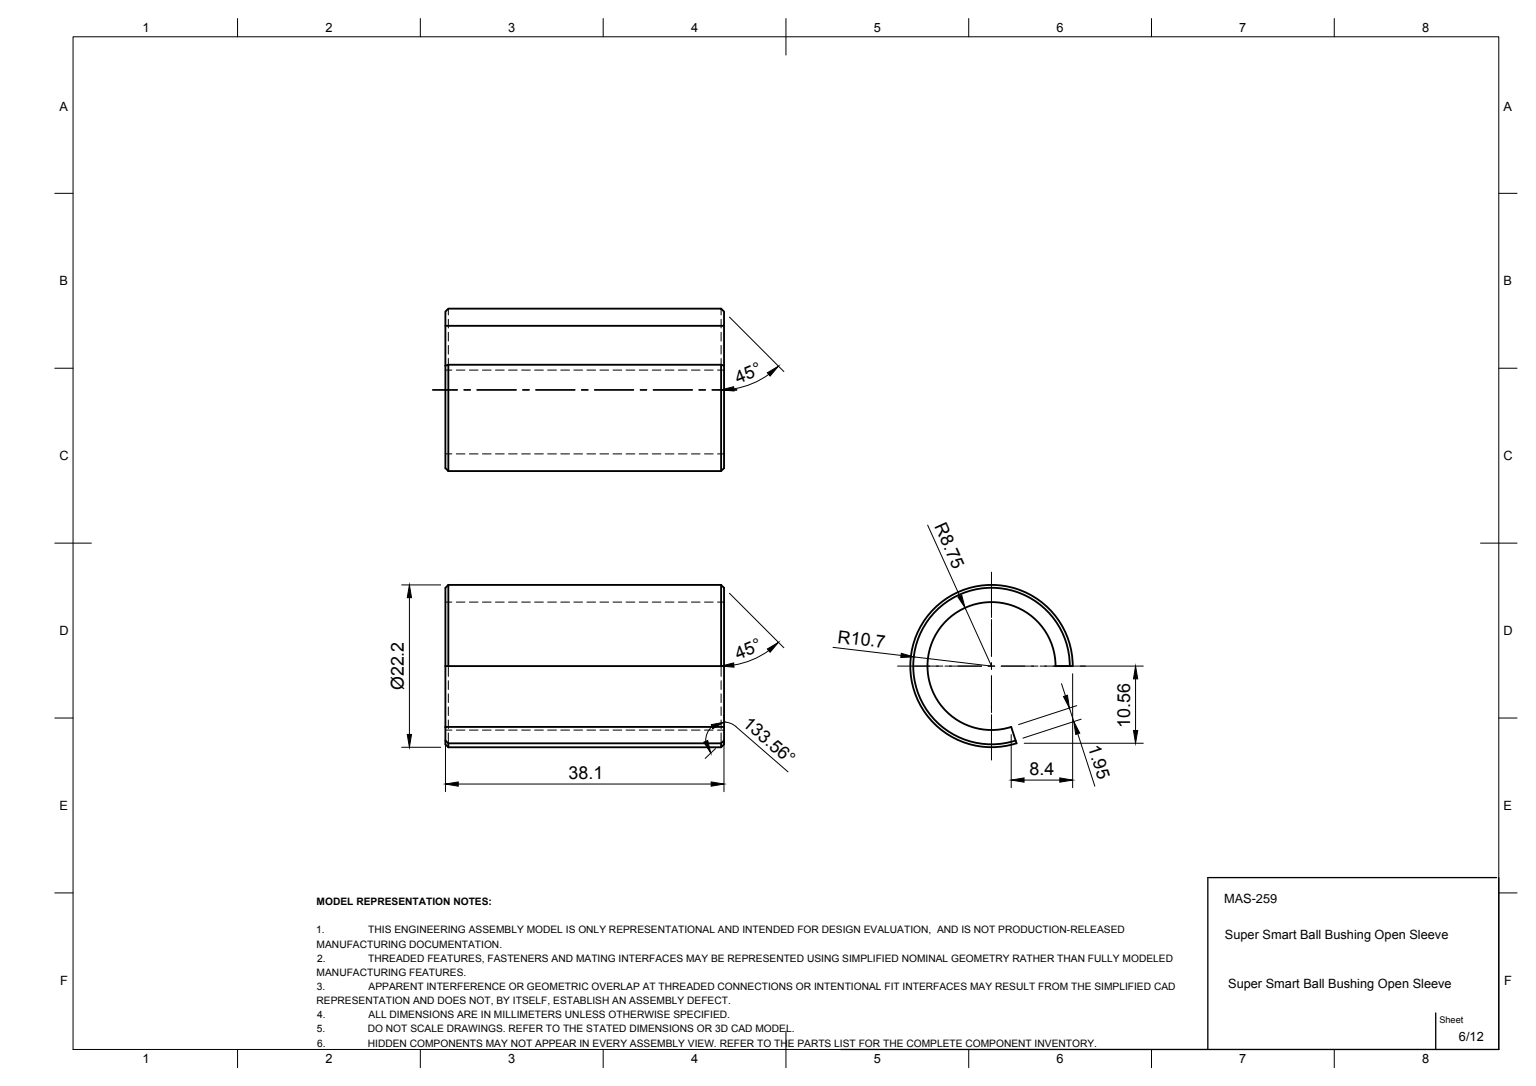
ISO-10303-21;
HEADER;
/* Generated by software containing ST-Developer
 * from STEP Tools, Inc. (www.steptools.com) 
 */

FILE_DESCRIPTION(
/* description */ (''),
/* implementation_level */ '2;1');

FILE_NAME(
/* name */ 'Super Smart Ball Bushing Open Sleeve.step',
/* time_stamp */ '2026-10-15T13:30:17-07:00',
/* author */ (''),
/* organization */ (''),
/* preprocessor_version */ 'ST-DEVELOPER v20.2',
/* originating_system */ 'Autodesk Translation Framework v15.15.0.0',
/* authorisation */ '');

FILE_SCHEMA (('AUTOMOTIVE_DESIGN { 1 0 10303 214 3 1 1 }'));
ENDSEC;

DATA;
#10=MECHANICAL_DESIGN_GEOMETRIC_PRESENTATION_REPRESENTATION('',(#1037),#71795);
#1017=SHAPE_REPRESENTATION_RELATIONSHIP('SRR','None',#72021,#1027);
#1027=ADVANCED_BREP_SHAPE_REPRESENTATION('',(#1047),#71789);
#1037=STYLED_ITEM('',(#72080),#1047);
#1047=MANIFOLD_SOLID_BREP('Body1',#13639);
#1092=CONICAL_SURFACE('',#14048,10.9,0.785398163397437);
#1093=CONICAL_SURFACE('',#14057,10.9,0.785398163397448);
#1624=PLANE('',#14046);
#1625=PLANE('',#14047);
#1626=PLANE('',#14051);
#1627=PLANE('',#14055);
#2178=FACE_OUTER_BOUND('',#2891,.T.);
#2179=FACE_OUTER_BOUND('',#2892,.T.);
#2180=FACE_OUTER_BOUND('',#2893,.T.);
#2181=FACE_OUTER_BOUND('',#2894,.T.);
#2182=FACE_OUTER_BOUND('',#2895,.T.);
#2183=FACE_OUTER_BOUND('',#2896,.T.);
#2184=FACE_OUTER_BOUND('',#2897,.T.);
#2185=FACE_OUTER_BOUND('',#2898,.T.);
#2891=EDGE_LOOP('',(#9677,#9678,#9679,#9680,#9681,#9682));
#2892=EDGE_LOOP('',(#9683,#9684,#9685,#9686,#9687,#9688));
#2893=EDGE_LOOP('',(#9689,#9690,#9691,#9692));
#2894=EDGE_LOOP('',(#9693,#9694,#9695,#9696));
#2895=EDGE_LOOP('',(#9697,#9698,#9699,#9700));
#2896=EDGE_LOOP('',(#9701,#9702,#9703,#9704));
#2897=EDGE_LOOP('',(#9705,#9706,#9707,#9708));
#2898=EDGE_LOOP('',(#9709,#9710,#9711,#9712));
#3531=CIRCLE('',#14049,10.7);
#3532=CIRCLE('',#14050,11.1);
#3533=CIRCLE('',#14052,8.75);
#3534=CIRCLE('',#14054,8.75);
#3535=CIRCLE('',#14056,10.7);
#3536=CIRCLE('',#14058,11.1);
#4023=LINE('',#19704,#4934);
#4024=LINE('',#19706,#4935);
#4025=LINE('',#19708,#4936);
#4026=LINE('',#19710,#4937);
#4027=LINE('',#19712,#4938);
#4028=LINE('',#19713,#4939);
#4029=LINE('',#19717,#4940);
#4030=LINE('',#19719,#4941);
#4031=LINE('',#19721,#4942);
#4032=LINE('',#19723,#4943);
#4033=LINE('',#19725,#4944);
#4034=LINE('',#19726,#4945);
#4934=VECTOR('',#15810,10.);
#4935=VECTOR('',#15811,10.);
#4936=VECTOR('',#15812,10.);
#4937=VECTOR('',#15813,10.);
#4938=VECTOR('',#15814,10.);
#4939=VECTOR('',#15815,10.);
#4940=VECTOR('',#15818,10.);
#4941=VECTOR('',#15819,10.);
#4942=VECTOR('',#15820,9.99999999999999);
#4943=VECTOR('',#15821,10.);
#4944=VECTOR('',#15822,10.);
#4945=VECTOR('',#15823,10.);
#5904=VERTEX_POINT('',#19702);
#5905=VERTEX_POINT('',#19703);
#5906=VERTEX_POINT('',#19705);
#5907=VERTEX_POINT('',#19707);
#5908=VERTEX_POINT('',#19709);
#5909=VERTEX_POINT('',#19711);
#5910=VERTEX_POINT('',#19715);
#5911=VERTEX_POINT('',#19716);
#5912=VERTEX_POINT('',#19718);
#5913=VERTEX_POINT('',#19720);
#5914=VERTEX_POINT('',#19722);
#5915=VERTEX_POINT('',#19724);
#7373=EDGE_CURVE('',#5904,#5905,#4023,.T.);
#7374=EDGE_CURVE('',#5906,#5904,#4024,.T.);
#7375=EDGE_CURVE('',#5907,#5906,#4025,.T.);
#7376=EDGE_CURVE('',#5908,#5907,#4026,.T.);
#7377=EDGE_CURVE('',#5909,#5908,#4027,.T.);
#7378=EDGE_CURVE('',#5905,#5909,#4028,.T.);
#7379=EDGE_CURVE('',#5910,#5911,#4029,.T.);
#7380=EDGE_CURVE('',#5912,#5910,#4030,.T.);
#7381=EDGE_CURVE('',#5913,#5912,#4031,.T.);
#7382=EDGE_CURVE('',#5914,#5913,#4032,.T.);
#7383=EDGE_CURVE('',#5915,#5914,#4033,.T.);
#7384=EDGE_CURVE('',#5911,#5915,#4034,.T.);
#7385=EDGE_CURVE('',#5904,#5911,#3531,.T.);
#7386=EDGE_CURVE('',#5905,#5910,#3532,.T.);
#7387=EDGE_CURVE('',#5906,#5915,#3533,.T.);
#7388=EDGE_CURVE('',#5907,#5914,#3534,.T.);
#7389=EDGE_CURVE('',#5908,#5913,#3535,.T.);
#7390=EDGE_CURVE('',#5909,#5912,#3536,.T.);
#9677=ORIENTED_EDGE('',*,*,#7373,.F.);
#9678=ORIENTED_EDGE('',*,*,#7374,.F.);
#9679=ORIENTED_EDGE('',*,*,#7375,.F.);
#9680=ORIENTED_EDGE('',*,*,#7376,.F.);
#9681=ORIENTED_EDGE('',*,*,#7377,.F.);
#9682=ORIENTED_EDGE('',*,*,#7378,.F.);
#9683=ORIENTED_EDGE('',*,*,#7379,.F.);
#9684=ORIENTED_EDGE('',*,*,#7380,.F.);
#9685=ORIENTED_EDGE('',*,*,#7381,.F.);
#9686=ORIENTED_EDGE('',*,*,#7382,.F.);
#9687=ORIENTED_EDGE('',*,*,#7383,.F.);
#9688=ORIENTED_EDGE('',*,*,#7384,.F.);
#9689=ORIENTED_EDGE('',*,*,#7379,.T.);
#9690=ORIENTED_EDGE('',*,*,#7385,.F.);
#9691=ORIENTED_EDGE('',*,*,#7373,.T.);
#9692=ORIENTED_EDGE('',*,*,#7386,.T.);
#9693=ORIENTED_EDGE('',*,*,#7384,.T.);
#9694=ORIENTED_EDGE('',*,*,#7387,.F.);
#9695=ORIENTED_EDGE('',*,*,#7374,.T.);
#9696=ORIENTED_EDGE('',*,*,#7385,.T.);
#9697=ORIENTED_EDGE('',*,*,#7383,.T.);
#9698=ORIENTED_EDGE('',*,*,#7388,.F.);
#9699=ORIENTED_EDGE('',*,*,#7375,.T.);
#9700=ORIENTED_EDGE('',*,*,#7387,.T.);
#9701=ORIENTED_EDGE('',*,*,#7382,.T.);
#9702=ORIENTED_EDGE('',*,*,#7389,.F.);
#9703=ORIENTED_EDGE('',*,*,#7376,.T.);
#9704=ORIENTED_EDGE('',*,*,#7388,.T.);
#9705=ORIENTED_EDGE('',*,*,#7381,.T.);
#9706=ORIENTED_EDGE('',*,*,#7390,.F.);
#9707=ORIENTED_EDGE('',*,*,#7377,.T.);
#9708=ORIENTED_EDGE('',*,*,#7389,.T.);
#9709=ORIENTED_EDGE('',*,*,#7380,.T.);
#9710=ORIENTED_EDGE('',*,*,#7386,.F.);
#9711=ORIENTED_EDGE('',*,*,#7378,.T.);
#9712=ORIENTED_EDGE('',*,*,#7390,.T.);
#12914=CYLINDRICAL_SURFACE('',#14053,8.75);
#12915=CYLINDRICAL_SURFACE('',#14059,11.1);
#13138=ADVANCED_FACE('',(#2178),#1624,.F.);
#13139=ADVANCED_FACE('',(#2179),#1625,.F.);
#13140=ADVANCED_FACE('',(#2180),#1092,.T.);
#13141=ADVANCED_FACE('',(#2181),#1626,.T.);
#13142=ADVANCED_FACE('',(#2182),#12914,.F.);
#13143=ADVANCED_FACE('',(#2183),#1627,.T.);
#13144=ADVANCED_FACE('',(#2184),#1093,.T.);
#13145=ADVANCED_FACE('',(#2185),#12915,.T.);
#13639=CLOSED_SHELL('',(#13138,#13139,#13140,#13141,#13142,#13143,#13144,
#13145));
#14045=AXIS2_PLACEMENT_3D('',#19700,#15806,#15807);
#14046=AXIS2_PLACEMENT_3D('',#19701,#15808,#15809);
#14047=AXIS2_PLACEMENT_3D('',#19714,#15816,#15817);
#14048=AXIS2_PLACEMENT_3D('',#19727,#15824,#15825);
#14049=AXIS2_PLACEMENT_3D('',#19728,#15826,#15827);
#14050=AXIS2_PLACEMENT_3D('',#19729,#15828,#15829);
#14051=AXIS2_PLACEMENT_3D('',#19730,#15830,#15831);
#14052=AXIS2_PLACEMENT_3D('',#19731,#15832,#15833);
#14053=AXIS2_PLACEMENT_3D('',#19732,#15834,#15835);
#14054=AXIS2_PLACEMENT_3D('',#19733,#15836,#15837);
#14055=AXIS2_PLACEMENT_3D('',#19734,#15838,#15839);
#14056=AXIS2_PLACEMENT_3D('',#19735,#15840,#15841);
#14057=AXIS2_PLACEMENT_3D('',#19736,#15842,#15843);
#14058=AXIS2_PLACEMENT_3D('',#19737,#15844,#15845);
#14059=AXIS2_PLACEMENT_3D('',#19738,#15846,#15847);
#15806=DIRECTION('axis',(0.,0.,1.));
#15807=DIRECTION('refdir',(1.,0.,0.));
#15808=DIRECTION('center_axis',(0.,0.987688340595138,-0.156434465040231));
#15809=DIRECTION('ref_axis',(0.,0.156434465040231,0.987688340595138));
#15810=DIRECTION('',(-0.707106781186555,-0.110615871041236,-0.698401123333703));
#15811=DIRECTION('',(0.,-0.156434465040231,-0.987688340595138));
#15812=DIRECTION('',(1.,0.,0.));
#15813=DIRECTION('',(0.,0.156434465040231,0.987688340595138));
#15814=DIRECTION('',(-0.707106781186547,0.110615871041237,0.698401123333711));
#15815=DIRECTION('',(-1.,0.,0.));
#15816=DIRECTION('center_axis',(0.,-0.156434465040231,0.987688340595138));
#15817=DIRECTION('ref_axis',(0.,-0.987688340595138,-0.156434465040231));
#15818=DIRECTION('',(0.707106781186555,0.698401123333703,0.110615871041236));
#15819=DIRECTION('',(1.,0.,0.));
#15820=DIRECTION('',(0.707106781186547,-0.69840112333371,-0.110615871041237));
#15821=DIRECTION('',(0.,-0.987688340595138,-0.156434465040231));
#15822=DIRECTION('',(-1.,0.,0.));
#15823=DIRECTION('',(0.,0.987688340595138,0.156434465040231));
#15824=DIRECTION('center_axis',(-1.,0.,0.));
#15825=DIRECTION('ref_axis',(0.,0.707106781186547,0.707106781186548));
#15826=DIRECTION('center_axis',(1.,0.,0.));
#15827=DIRECTION('ref_axis',(0.,0.,-1.));
#15828=DIRECTION('center_axis',(1.,0.,0.));
#15829=DIRECTION('ref_axis',(0.,0.,-1.));
#15830=DIRECTION('center_axis',(1.,0.,0.));
#15831=DIRECTION('ref_axis',(0.,0.,-1.));
#15832=DIRECTION('center_axis',(1.,0.,0.));
#15833=DIRECTION('ref_axis',(0.,0.,-1.));
#15834=DIRECTION('center_axis',(1.,0.,0.));
#15835=DIRECTION('ref_axis',(0.,0.707106781186547,0.707106781186548));
#15836=DIRECTION('center_axis',(1.,0.,0.));
#15837=DIRECTION('ref_axis',(0.,0.,-1.));
#15838=DIRECTION('center_axis',(-1.,0.,0.));
#15839=DIRECTION('ref_axis',(0.,0.,1.));
#15840=DIRECTION('center_axis',(1.,0.,0.));
#15841=DIRECTION('ref_axis',(0.,0.,-1.));
#15842=DIRECTION('center_axis',(1.,0.,0.));
#15843=DIRECTION('ref_axis',(0.,0.707106781186547,0.707106781186548));
#15844=DIRECTION('center_axis',(1.,0.,0.));
#15845=DIRECTION('ref_axis',(0.,0.,-1.));
#15846=DIRECTION('center_axis',(1.,0.,0.));
#15847=DIRECTION('ref_axis',(0.,0.707106781186547,0.707106781186548));
#19700=CARTESIAN_POINT('',(0.,0.,0.));
#19701=CARTESIAN_POINT('Origin',(32.85,20.175708507973,25.1612827382037));
#19702=CARTESIAN_POINT('',(70.95,20.5511512240695,27.5317347556321));
#19703=CARTESIAN_POINT('',(70.55,20.4885774380534,27.136659419394));
#19704=CARTESIAN_POINT('',(70.75,20.5198643310615,27.334197087513));
#19705=CARTESIAN_POINT('',(70.95,20.856198430898,29.4577270197926));
#19706=CARTESIAN_POINT('',(70.95,21.3074181245908,32.306616044297));
#19707=CARTESIAN_POINT('',(32.85,20.856198430898,29.4577270197926));
#19708=CARTESIAN_POINT('',(51.9,20.856198430898,29.4577270197926));
#19709=CARTESIAN_POINT('',(32.85,20.5511512240695,27.531734755632));
#19710=CARTESIAN_POINT('',(32.85,21.3312780728969,32.4572618290548));
#19711=CARTESIAN_POINT('',(33.25,20.4885774380534,27.136659419394));
#19712=CARTESIAN_POINT('',(33.05,20.5198643310615,27.334197087513));
#19713=CARTESIAN_POINT('',(51.9,20.4885774380534,27.136659419394));
#19714=CARTESIAN_POINT('Origin',(32.85,22.225,38.1));
#19715=CARTESIAN_POINT('',(70.55,11.261659419394,36.3635774380534));
#19716=CARTESIAN_POINT('',(70.95,11.6567347556321,36.4261512240695));
#19717=CARTESIAN_POINT('',(70.75,11.459197087513,36.3948643310615));
#19718=CARTESIAN_POINT('',(33.25,11.261659419394,36.3635774380534));
#19719=CARTESIAN_POINT('',(51.9,11.261659419394,36.3635774380534));
#19720=CARTESIAN_POINT('',(32.85,11.656734755632,36.4261512240695));
#19721=CARTESIAN_POINT('',(33.05,11.459197087513,36.3948643310615));
#19722=CARTESIAN_POINT('',(32.85,13.5827270197925,36.731198430898));
#19723=CARTESIAN_POINT('',(32.85,27.4440761810895,38.926620459953));
#19724=CARTESIAN_POINT('',(70.95,13.5827270197925,36.731198430898));
#19725=CARTESIAN_POINT('',(51.9,13.5827270197925,36.731198430898));
#19726=CARTESIAN_POINT('',(70.95,26.4929361293956,38.7759746751952));
#19727=CARTESIAN_POINT('Origin',(70.75,22.225,38.1));
#19728=CARTESIAN_POINT('Origin',(70.95,22.225,38.1));
#19729=CARTESIAN_POINT('Origin',(70.55,22.225,38.1));
#19730=CARTESIAN_POINT('Origin',(70.95,30.975,38.1));
#19731=CARTESIAN_POINT('Origin',(70.95,22.225,38.1));
#19732=CARTESIAN_POINT('Origin',(51.9,22.225,38.1));
#19733=CARTESIAN_POINT('Origin',(32.85,22.225,38.1));
#19734=CARTESIAN_POINT('Origin',(32.85,32.925,38.1));
#19735=CARTESIAN_POINT('Origin',(32.85,22.225,38.1));
#19736=CARTESIAN_POINT('Origin',(33.05,22.225,38.1));
#19737=CARTESIAN_POINT('Origin',(33.25,22.225,38.1));
#19738=CARTESIAN_POINT('Origin',(51.9,22.225,38.1));
#71777=UNCERTAINTY_MEASURE_WITH_UNIT(LENGTH_MEASURE(0.01),#71796,
'DISTANCE_ACCURACY_VALUE',
'Maximum model space distance between geometric entities at asserted c
onnectivities');
#71783=UNCERTAINTY_MEASURE_WITH_UNIT(LENGTH_MEASURE(0.01),#71796,
'DISTANCE_ACCURACY_VALUE',
'Maximum model space distance between geometric entities at asserted c
onnectivities');
#71789=(
GEOMETRIC_REPRESENTATION_CONTEXT(3)
GLOBAL_UNCERTAINTY_ASSIGNED_CONTEXT((#71777))
GLOBAL_UNIT_ASSIGNED_CONTEXT((#71796,#71798,#71799))
REPRESENTATION_CONTEXT('','3D')
);
#71795=(
GEOMETRIC_REPRESENTATION_CONTEXT(3)
GLOBAL_UNCERTAINTY_ASSIGNED_CONTEXT((#71783))
GLOBAL_UNIT_ASSIGNED_CONTEXT((#71796,#71798,#71799))
REPRESENTATION_CONTEXT('','3D')
);
#71796=(
LENGTH_UNIT()
NAMED_UNIT(*)
SI_UNIT(.MILLI.,.METRE.)
);
#71798=(
NAMED_UNIT(*)
PLANE_ANGLE_UNIT()
SI_UNIT($,.RADIAN.)
);
#71799=(
NAMED_UNIT(*)
SI_UNIT($,.STERADIAN.)
SOLID_ANGLE_UNIT()
);
#71805=SHAPE_DEFINITION_REPRESENTATION(#71816,#72021);
#71816=PRODUCT_DEFINITION_SHAPE('',$,#72033);
#72021=SHAPE_REPRESENTATION('',(#14045),#71789);
#72027=PRODUCT_DEFINITION_CONTEXT('part definition',#72062,'design');
#72033=PRODUCT_DEFINITION('Super Smart Ball Bushing Open Sleeve',
'Super Smart Ball Bushing Open Sleeve',#72044,#72027);
#72044=PRODUCT_DEFINITION_FORMATION('',$,#72069);
#72062=APPLICATION_CONTEXT(
'Core Data for Automotive Mechanical Design Process');
#72063=PRODUCT_CONTEXT('part definition',#72062,'mechanical');
#72069=PRODUCT('Super Smart Ball Bushing Open Sleeve',
'Super Smart Ball Bushing Open Sleeve',$,(#72063));
#72080=PRESENTATION_STYLE_ASSIGNMENT((#72091));
#72091=SURFACE_STYLE_USAGE(.BOTH.,#72102);
#72102=SURFACE_SIDE_STYLE('',(#72113));
#72113=SURFACE_STYLE_FILL_AREA(#72124);
#72124=FILL_AREA_STYLE('Opaque(226,229,233)',(#72135));
#72135=FILL_AREA_STYLE_COLOUR('Opaque(226,229,233)',#72146);
#72146=COLOUR_RGB('Opaque(226,229,233)', 0.72549020, 0.75294118, 0.79215686);
ENDSEC;
END-ISO-10303-21;
